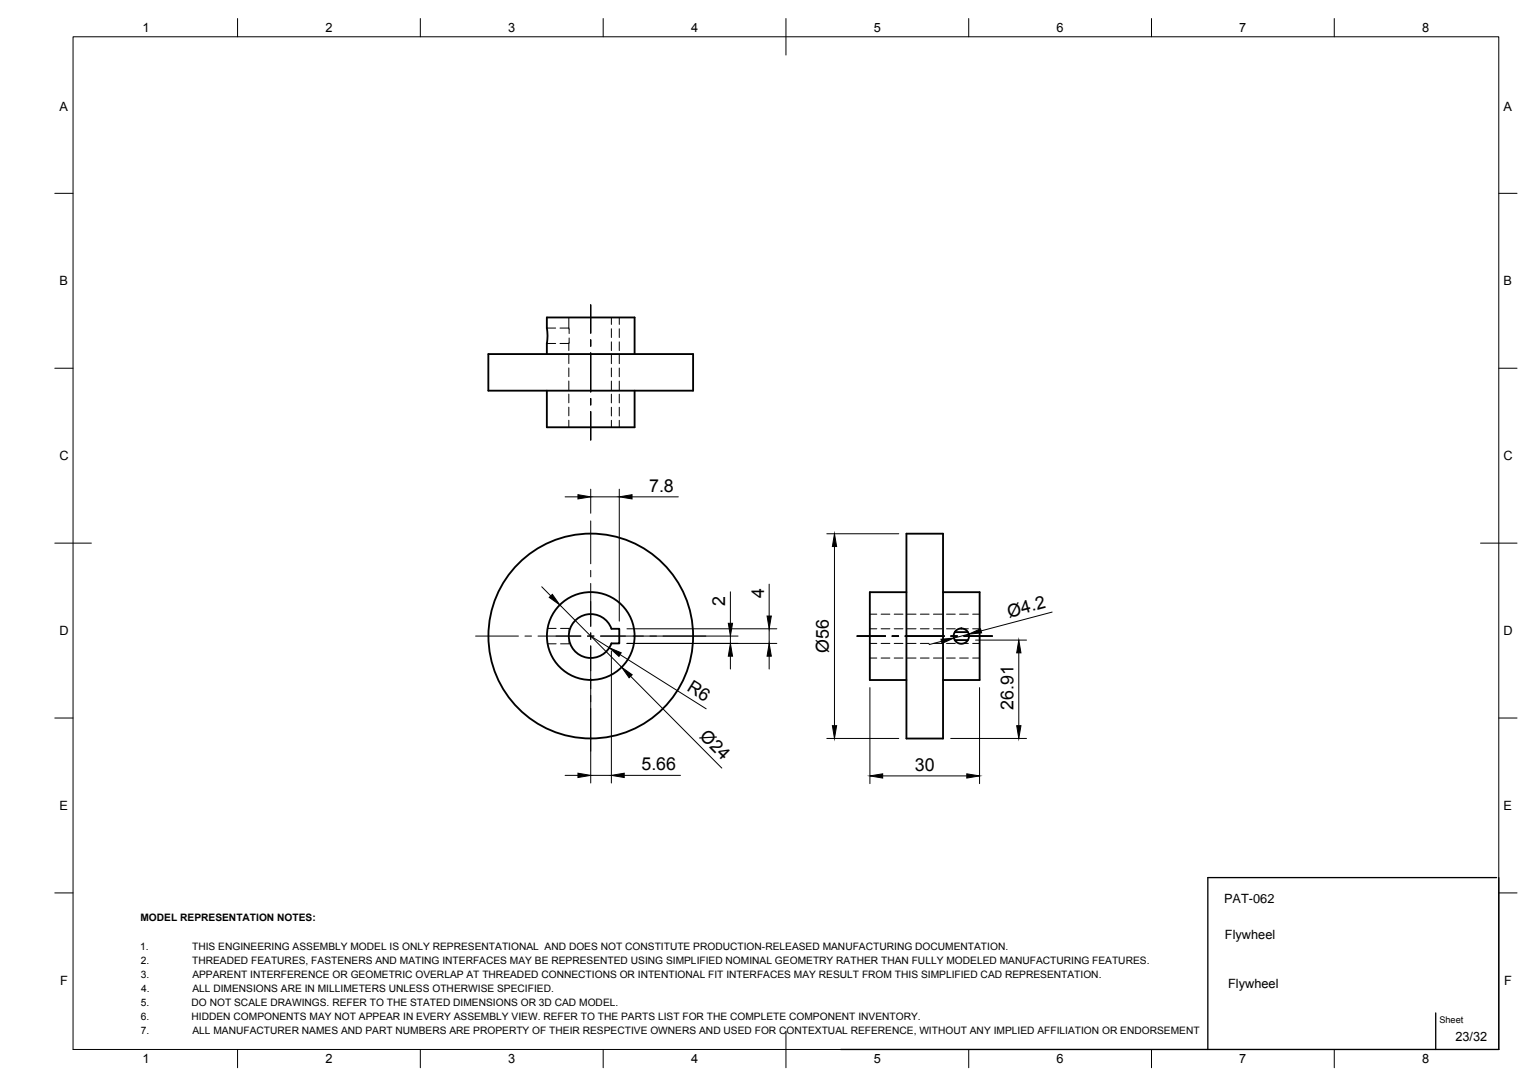
ISO-10303-21;
HEADER;
/* Generated by software containing ST-Developer
 * from STEP Tools, Inc. (www.steptools.com) 
 */

FILE_DESCRIPTION(
/* description */ ('Jaw-coupled motor to shaft test stand'),
/* implementation_level */ '2;1');

FILE_NAME(
/* name */ 'Flywheel.step',
/* time_stamp */ '2026-10-27T10:46:06-07:00',
/* author */ (''),
/* organization */ (''),
/* preprocessor_version */ 'ST-DEVELOPER v20.2',
/* originating_system */ 'Autodesk Translation Framework v15.17.0.0',
/* authorisation */ '');

FILE_SCHEMA (('AUTOMOTIVE_DESIGN { 1 0 10303 214 3 1 1 }'));
ENDSEC;

DATA;
#10=MECHANICAL_DESIGN_GEOMETRIC_PRESENTATION_REPRESENTATION('',(#362),#19361);
#255=B_SPLINE_CURVE_WITH_KNOTS('',3,(#16957,#16958,#16959,#16960,#16961,
#16962,#16963,#16964,#16965,#16966),.UNSPECIFIED.,.F.,.F.,(4,2,2,2,4),(0.847831445683403,
0.87827457693095,0.958092875386316,1.03791117384168,1.06835430508923),
 .UNSPECIFIED.);
#256=B_SPLINE_CURVE_WITH_KNOTS('',3,(#16972,#16973,#16974,#16975,#16976,
#16977,#16978,#16979,#16980,#16981,#16982,#16983,#16984,#16985,#16986,#16987,
#16988,#16989),.UNSPECIFIED.,.F.,.F.,(4,2,2,2,2,2,2,2,4),(0.,0.0792812130427884,
0.158562426085577,0.237841058284634,0.317119690483692,0.396398322682749,
0.475676954881807,0.554958167924595,0.634239380967384),.UNSPECIFIED.);
#257=B_SPLINE_CURVE_WITH_KNOTS('',3,(#16990,#16991,#16992,#16993,#16994,
#16995,#16996,#16997,#16998,#16999,#17000,#17001,#17002,#17003,#17004,#17005,
#17006,#17007),.UNSPECIFIED.,.F.,.F.,(4,2,2,2,2,2,2,2,4),(0.634239380967384,
0.713520594010172,0.792801807052961,0.872080439252018,0.951359071451076,
1.03063770365013,1.10991633584919,1.18919754889198,1.26847876193477),
 .UNSPECIFIED.);
#258=B_SPLINE_CURVE_WITH_KNOTS('',3,(#17010,#17011,#17012,#17013,#17014,
#17015,#17016,#17017,#17018,#17019),.UNSPECIFIED.,.F.,.F.,(4,2,2,2,4),(0.209102862092526,
0.239545993340073,0.319364291795439,0.399182590250804,0.429625721498351),
 .UNSPECIFIED.);
#297=SHAPE_REPRESENTATION_RELATIONSHIP('SRR','None',#19513,#329);
#329=ADVANCED_BREP_SHAPE_REPRESENTATION('',(#393),#19349);
#362=STYLED_ITEM('',(#19760),#393);
#393=MANIFOLD_SOLID_BREP('Body1',#11008);
#489=FACE_BOUND('',#1956,.T.);
#490=FACE_BOUND('',#1958,.T.);
#491=FACE_BOUND('',#1960,.T.);
#492=FACE_BOUND('',#1962,.T.);
#493=FACE_BOUND('',#1965,.T.);
#494=FACE_BOUND('',#1968,.T.);
#666=PLANE('',#11782);
#667=PLANE('',#11787);
#668=PLANE('',#11788);
#669=PLANE('',#11789);
#670=PLANE('',#11790);
#671=PLANE('',#11791);
#672=PLANE('',#11796);
#673=PLANE('',#11799);
#674=PLANE('',#11806);
#1243=FACE_OUTER_BOUND('',#1949,.T.);
#1244=FACE_OUTER_BOUND('',#1950,.T.);
#1245=FACE_OUTER_BOUND('',#1951,.T.);
#1246=FACE_OUTER_BOUND('',#1952,.T.);
#1247=FACE_OUTER_BOUND('',#1953,.T.);
#1248=FACE_OUTER_BOUND('',#1954,.T.);
#1249=FACE_OUTER_BOUND('',#1955,.T.);
#1250=FACE_OUTER_BOUND('',#1957,.T.);
#1251=FACE_OUTER_BOUND('',#1959,.T.);
#1252=FACE_OUTER_BOUND('',#1961,.T.);
#1253=FACE_OUTER_BOUND('',#1963,.T.);
#1254=FACE_OUTER_BOUND('',#1964,.T.);
#1255=FACE_OUTER_BOUND('',#1966,.T.);
#1256=FACE_OUTER_BOUND('',#1967,.T.);
#1949=EDGE_LOOP('',(#8286,#8287));
#1950=EDGE_LOOP('',(#8288,#8289,#8290,#8291,#8292,#8293,#8294,#8295,#8296));
#1951=EDGE_LOOP('',(#8297,#8298,#8299));
#1952=EDGE_LOOP('',(#8300,#8301,#8302,#8303));
#1953=EDGE_LOOP('',(#8304,#8305,#8306,#8307));
#1954=EDGE_LOOP('',(#8308,#8309,#8310,#8311));
#1955=EDGE_LOOP('',(#8312));
#1956=EDGE_LOOP('',(#8313,#8314,#8315,#8316));
#1957=EDGE_LOOP('',(#8317,#8318,#8319,#8320));
#1958=EDGE_LOOP('',(#8321,#8322,#8323,#8324));
#1959=EDGE_LOOP('',(#8325));
#1960=EDGE_LOOP('',(#8326));
#1961=EDGE_LOOP('',(#8327));
#1962=EDGE_LOOP('',(#8328));
#1963=EDGE_LOOP('',(#8329,#8330,#8331,#8332));
#1964=EDGE_LOOP('',(#8333,#8334,#8335,#8336));
#1965=EDGE_LOOP('',(#8337,#8338));
#1966=EDGE_LOOP('',(#8339,#8340,#8341,#8342));
#1967=EDGE_LOOP('',(#8343));
#1968=EDGE_LOOP('',(#8344,#8345,#8346,#8347));
#2682=LINE('',#16953,#3835);
#2683=LINE('',#16970,#3836);
#2684=LINE('',#17021,#3837);
#2685=LINE('',#17025,#3838);
#2686=LINE('',#17027,#3839);
#2687=LINE('',#17029,#3840);
#2688=LINE('',#17030,#3841);
#2689=LINE('',#17033,#3842);
#2690=LINE('',#17035,#3843);
#2691=LINE('',#17036,#3844);
#2692=LINE('',#17039,#3845);
#2693=LINE('',#17041,#3846);
#2694=LINE('',#17042,#3847);
#2695=LINE('',#17060,#3848);
#2696=LINE('',#17063,#3849);
#2697=LINE('',#17066,#3850);
#3835=VECTOR('',#13467,1.);
#3836=VECTOR('',#13474,0.21);
#3837=VECTOR('',#13479,1.);
#3838=VECTOR('',#13482,1.);
#3839=VECTOR('',#13483,1.);
#3840=VECTOR('',#13484,1.);
#3841=VECTOR('',#13485,1.);
#3842=VECTOR('',#13488,1.);
#3843=VECTOR('',#13489,1.);
#3844=VECTOR('',#13490,1.);
#3845=VECTOR('',#13493,1.);
#3846=VECTOR('',#13494,1.);
#3847=VECTOR('',#13495,1.);
#3848=VECTOR('',#13520,2.8);
#3849=VECTOR('',#13523,1.2);
#3850=VECTOR('',#13528,1.2);
#4816=CIRCLE('',#11783,0.21);
#4817=CIRCLE('',#11785,0.21);
#4818=CIRCLE('',#11786,0.21);
#4819=CIRCLE('',#11792,1.2);
#4820=CIRCLE('',#11793,0.6);
#4821=CIRCLE('',#11795,0.6);
#4822=CIRCLE('',#11797,2.8);
#4823=CIRCLE('',#11798,1.2);
#4824=CIRCLE('',#11800,2.8);
#4825=CIRCLE('',#11801,1.2);
#4826=CIRCLE('',#11804,1.2);
#5262=VERTEX_POINT('',#16951);
#5263=VERTEX_POINT('',#16952);
#5264=VERTEX_POINT('',#16956);
#5265=VERTEX_POINT('',#16967);
#5266=VERTEX_POINT('',#16969);
#5267=VERTEX_POINT('',#16971);
#5268=VERTEX_POINT('',#17008);
#5269=VERTEX_POINT('',#17023);
#5270=VERTEX_POINT('',#17024);
#5271=VERTEX_POINT('',#17026);
#5272=VERTEX_POINT('',#17028);
#5273=VERTEX_POINT('',#17032);
#5274=VERTEX_POINT('',#17034);
#5275=VERTEX_POINT('',#17038);
#5276=VERTEX_POINT('',#17040);
#5277=VERTEX_POINT('',#17044);
#5278=VERTEX_POINT('',#17050);
#5279=VERTEX_POINT('',#17052);
#5280=VERTEX_POINT('',#17055);
#5281=VERTEX_POINT('',#17057);
#5282=VERTEX_POINT('',#17062);
#6354=EDGE_CURVE('',#5262,#5263,#2682,.T.);
#6355=EDGE_CURVE('',#5262,#5263,#4816,.T.);
#6356=EDGE_CURVE('',#5264,#5262,#255,.T.);
#6357=EDGE_CURVE('',#5265,#5264,#4817,.T.);
#6358=EDGE_CURVE('',#5265,#5266,#2683,.T.);
#6359=EDGE_CURVE('',#5267,#5266,#256,.T.);
#6360=EDGE_CURVE('',#5266,#5267,#257,.T.);
#6361=EDGE_CURVE('',#5268,#5265,#4818,.T.);
#6362=EDGE_CURVE('',#5263,#5268,#258,.T.);
#6363=EDGE_CURVE('',#5268,#5264,#2684,.T.);
#6364=EDGE_CURVE('',#5269,#5270,#2685,.T.);
#6365=EDGE_CURVE('',#5269,#5271,#2686,.T.);
#6366=EDGE_CURVE('',#5272,#5271,#2687,.T.);
#6367=EDGE_CURVE('',#5270,#5272,#2688,.T.);
#6368=EDGE_CURVE('',#5273,#5269,#2689,.T.);
#6369=EDGE_CURVE('',#5273,#5274,#2690,.T.);
#6370=EDGE_CURVE('',#5271,#5274,#2691,.T.);
#6371=EDGE_CURVE('',#5275,#5273,#2692,.T.);
#6372=EDGE_CURVE('',#5276,#5275,#2693,.T.);
#6373=EDGE_CURVE('',#5274,#5276,#2694,.T.);
#6374=EDGE_CURVE('',#5277,#5277,#4819,.T.);
#6375=EDGE_CURVE('',#5276,#5272,#4820,.T.);
#6376=EDGE_CURVE('',#5275,#5270,#4821,.T.);
#6377=EDGE_CURVE('',#5278,#5278,#4822,.T.);
#6378=EDGE_CURVE('',#5279,#5279,#4823,.T.);
#6379=EDGE_CURVE('',#5280,#5280,#4824,.T.);
#6380=EDGE_CURVE('',#5281,#5281,#4825,.T.);
#6381=EDGE_CURVE('',#5278,#5280,#2695,.T.);
#6382=EDGE_CURVE('',#5281,#5282,#2696,.T.);
#6383=EDGE_CURVE('',#5282,#5282,#4826,.T.);
#6384=EDGE_CURVE('',#5277,#5279,#2697,.T.);
#8286=ORIENTED_EDGE('',*,*,#6354,.F.);
#8287=ORIENTED_EDGE('',*,*,#6355,.T.);
#8288=ORIENTED_EDGE('',*,*,#6356,.F.);
#8289=ORIENTED_EDGE('',*,*,#6357,.F.);
#8290=ORIENTED_EDGE('',*,*,#6358,.T.);
#8291=ORIENTED_EDGE('',*,*,#6359,.F.);
#8292=ORIENTED_EDGE('',*,*,#6360,.F.);
#8293=ORIENTED_EDGE('',*,*,#6358,.F.);
#8294=ORIENTED_EDGE('',*,*,#6361,.F.);
#8295=ORIENTED_EDGE('',*,*,#6362,.F.);
#8296=ORIENTED_EDGE('',*,*,#6355,.F.);
#8297=ORIENTED_EDGE('',*,*,#6363,.F.);
#8298=ORIENTED_EDGE('',*,*,#6361,.T.);
#8299=ORIENTED_EDGE('',*,*,#6357,.T.);
#8300=ORIENTED_EDGE('',*,*,#6364,.F.);
#8301=ORIENTED_EDGE('',*,*,#6365,.T.);
#8302=ORIENTED_EDGE('',*,*,#6366,.F.);
#8303=ORIENTED_EDGE('',*,*,#6367,.F.);
#8304=ORIENTED_EDGE('',*,*,#6368,.F.);
#8305=ORIENTED_EDGE('',*,*,#6369,.T.);
#8306=ORIENTED_EDGE('',*,*,#6370,.F.);
#8307=ORIENTED_EDGE('',*,*,#6365,.F.);
#8308=ORIENTED_EDGE('',*,*,#6371,.F.);
#8309=ORIENTED_EDGE('',*,*,#6372,.F.);
#8310=ORIENTED_EDGE('',*,*,#6373,.F.);
#8311=ORIENTED_EDGE('',*,*,#6369,.F.);
#8312=ORIENTED_EDGE('',*,*,#6374,.T.);
#8313=ORIENTED_EDGE('',*,*,#6366,.T.);
#8314=ORIENTED_EDGE('',*,*,#6370,.T.);
#8315=ORIENTED_EDGE('',*,*,#6373,.T.);
#8316=ORIENTED_EDGE('',*,*,#6375,.T.);
#8317=ORIENTED_EDGE('',*,*,#6367,.T.);
#8318=ORIENTED_EDGE('',*,*,#6375,.F.);
#8319=ORIENTED_EDGE('',*,*,#6372,.T.);
#8320=ORIENTED_EDGE('',*,*,#6376,.T.);
#8321=ORIENTED_EDGE('',*,*,#6362,.T.);
#8322=ORIENTED_EDGE('',*,*,#6363,.T.);
#8323=ORIENTED_EDGE('',*,*,#6356,.T.);
#8324=ORIENTED_EDGE('',*,*,#6354,.T.);
#8325=ORIENTED_EDGE('',*,*,#6377,.T.);
#8326=ORIENTED_EDGE('',*,*,#6378,.F.);
#8327=ORIENTED_EDGE('',*,*,#6379,.F.);
#8328=ORIENTED_EDGE('',*,*,#6380,.F.);
#8329=ORIENTED_EDGE('',*,*,#6377,.F.);
#8330=ORIENTED_EDGE('',*,*,#6381,.T.);
#8331=ORIENTED_EDGE('',*,*,#6379,.T.);
#8332=ORIENTED_EDGE('',*,*,#6381,.F.);
#8333=ORIENTED_EDGE('',*,*,#6380,.T.);
#8334=ORIENTED_EDGE('',*,*,#6382,.T.);
#8335=ORIENTED_EDGE('',*,*,#6383,.T.);
#8336=ORIENTED_EDGE('',*,*,#6382,.F.);
#8337=ORIENTED_EDGE('',*,*,#6359,.T.);
#8338=ORIENTED_EDGE('',*,*,#6360,.T.);
#8339=ORIENTED_EDGE('',*,*,#6374,.F.);
#8340=ORIENTED_EDGE('',*,*,#6384,.T.);
#8341=ORIENTED_EDGE('',*,*,#6378,.T.);
#8342=ORIENTED_EDGE('',*,*,#6384,.F.);
#8343=ORIENTED_EDGE('',*,*,#6383,.F.);
#8344=ORIENTED_EDGE('',*,*,#6364,.T.);
#8345=ORIENTED_EDGE('',*,*,#6376,.F.);
#8346=ORIENTED_EDGE('',*,*,#6371,.T.);
#8347=ORIENTED_EDGE('',*,*,#6368,.T.);
#10333=CYLINDRICAL_SURFACE('',#11784,0.21);
#10334=CYLINDRICAL_SURFACE('',#11794,0.6);
#10335=CYLINDRICAL_SURFACE('',#11802,2.8);
#10336=CYLINDRICAL_SURFACE('',#11803,1.2);
#10337=CYLINDRICAL_SURFACE('',#11805,1.2);
#10585=ADVANCED_FACE('',(#1243),#666,.T.);
#10586=ADVANCED_FACE('',(#1244),#10333,.F.);
#10587=ADVANCED_FACE('',(#1245),#667,.T.);
#10588=ADVANCED_FACE('',(#1246),#668,.F.);
#10589=ADVANCED_FACE('',(#1247),#669,.F.);
#10590=ADVANCED_FACE('',(#1248),#670,.F.);
#10591=ADVANCED_FACE('',(#1249,#489),#671,.T.);
#10592=ADVANCED_FACE('',(#1250,#490),#10334,.F.);
#10593=ADVANCED_FACE('',(#1251,#491),#672,.T.);
#10594=ADVANCED_FACE('',(#1252,#492),#673,.F.);
#10595=ADVANCED_FACE('',(#1253),#10335,.T.);
#10596=ADVANCED_FACE('',(#1254,#493),#10336,.T.);
#10597=ADVANCED_FACE('',(#1255),#10337,.T.);
#10598=ADVANCED_FACE('',(#1256,#494),#674,.F.);
#11008=CLOSED_SHELL('',(#10585,#10586,#10587,#10588,#10589,#10590,#10591,
#10592,#10593,#10594,#10595,#10596,#10597,#10598));
#11781=AXIS2_PLACEMENT_3D('',#16949,#13463,#13464);
#11782=AXIS2_PLACEMENT_3D('',#16950,#13465,#13466);
#11783=AXIS2_PLACEMENT_3D('',#16954,#13468,#13469);
#11784=AXIS2_PLACEMENT_3D('',#16955,#13470,#13471);
#11785=AXIS2_PLACEMENT_3D('',#16968,#13472,#13473);
#11786=AXIS2_PLACEMENT_3D('',#17009,#13475,#13476);
#11787=AXIS2_PLACEMENT_3D('',#17020,#13477,#13478);
#11788=AXIS2_PLACEMENT_3D('',#17022,#13480,#13481);
#11789=AXIS2_PLACEMENT_3D('',#17031,#13486,#13487);
#11790=AXIS2_PLACEMENT_3D('',#17037,#13491,#13492);
#11791=AXIS2_PLACEMENT_3D('',#17043,#13496,#13497);
#11792=AXIS2_PLACEMENT_3D('',#17045,#13498,#13499);
#11793=AXIS2_PLACEMENT_3D('',#17046,#13500,#13501);
#11794=AXIS2_PLACEMENT_3D('',#17047,#13502,#13503);
#11795=AXIS2_PLACEMENT_3D('',#17048,#13504,#13505);
#11796=AXIS2_PLACEMENT_3D('',#17049,#13506,#13507);
#11797=AXIS2_PLACEMENT_3D('',#17051,#13508,#13509);
#11798=AXIS2_PLACEMENT_3D('',#17053,#13510,#13511);
#11799=AXIS2_PLACEMENT_3D('',#17054,#13512,#13513);
#11800=AXIS2_PLACEMENT_3D('',#17056,#13514,#13515);
#11801=AXIS2_PLACEMENT_3D('',#17058,#13516,#13517);
#11802=AXIS2_PLACEMENT_3D('',#17059,#13518,#13519);
#11803=AXIS2_PLACEMENT_3D('',#17061,#13521,#13522);
#11804=AXIS2_PLACEMENT_3D('',#17064,#13524,#13525);
#11805=AXIS2_PLACEMENT_3D('',#17065,#13526,#13527);
#11806=AXIS2_PLACEMENT_3D('',#17067,#13529,#13530);
#13463=DIRECTION('axis',(0.,0.,1.));
#13464=DIRECTION('refdir',(1.,0.,0.));
#13465=DIRECTION('center_axis',(0.,0.,1.));
#13466=DIRECTION('ref_axis',(1.,0.,0.));
#13467=DIRECTION('',(0.,1.,0.));
#13468=DIRECTION('center_axis',(0.,0.,1.));
#13469=DIRECTION('ref_axis',(1.,0.,0.));
#13470=DIRECTION('center_axis',(0.,0.,1.));
#13471=DIRECTION('ref_axis',(1.,0.,0.));
#13472=DIRECTION('center_axis',(0.,0.,1.));
#13473=DIRECTION('ref_axis',(1.,0.,0.));
#13474=DIRECTION('',(0.,0.,1.));
#13475=DIRECTION('center_axis',(0.,0.,1.));
#13476=DIRECTION('ref_axis',(1.,0.,0.));
#13477=DIRECTION('center_axis',(0.,0.,1.));
#13478=DIRECTION('ref_axis',(1.,0.,0.));
#13479=DIRECTION('',(0.,-1.,0.));
#13480=DIRECTION('center_axis',(-1.,0.,0.));
#13481=DIRECTION('ref_axis',(0.,0.,1.));
#13482=DIRECTION('',(0.,0.,1.));
#13483=DIRECTION('',(0.,1.,0.));
#13484=DIRECTION('',(0.,0.,-1.));
#13485=DIRECTION('',(0.,1.,0.));
#13486=DIRECTION('center_axis',(0.,0.,-1.));
#13487=DIRECTION('ref_axis',(-1.,0.,0.));
#13488=DIRECTION('',(-1.,0.,0.));
#13489=DIRECTION('',(0.,1.,0.));
#13490=DIRECTION('',(1.,0.,0.));
#13491=DIRECTION('center_axis',(1.,0.,0.));
#13492=DIRECTION('ref_axis',(0.,0.,-1.));
#13493=DIRECTION('',(0.,0.,-1.));
#13494=DIRECTION('',(0.,-1.,0.));
#13495=DIRECTION('',(0.,0.,1.));
#13496=DIRECTION('center_axis',(0.,1.,0.));
#13497=DIRECTION('ref_axis',(1.,0.,0.));
#13498=DIRECTION('center_axis',(0.,1.,0.));
#13499=DIRECTION('ref_axis',(1.,0.,0.));
#13500=DIRECTION('center_axis',(0.,-1.,0.));
#13501=DIRECTION('ref_axis',(1.,0.,0.));
#13502=DIRECTION('center_axis',(0.,1.,0.));
#13503=DIRECTION('ref_axis',(-1.83697019872103E-16,0.,1.));
#13504=DIRECTION('center_axis',(0.,-1.,0.));
#13505=DIRECTION('ref_axis',(1.,0.,0.));
#13506=DIRECTION('center_axis',(0.,1.,0.));
#13507=DIRECTION('ref_axis',(1.,0.,0.));
#13508=DIRECTION('center_axis',(0.,1.,0.));
#13509=DIRECTION('ref_axis',(1.,0.,0.));
#13510=DIRECTION('center_axis',(0.,1.,0.));
#13511=DIRECTION('ref_axis',(1.,0.,0.));
#13512=DIRECTION('center_axis',(0.,1.,0.));
#13513=DIRECTION('ref_axis',(1.,0.,0.));
#13514=DIRECTION('center_axis',(0.,1.,0.));
#13515=DIRECTION('ref_axis',(1.,0.,0.));
#13516=DIRECTION('center_axis',(0.,-1.,0.));
#13517=DIRECTION('ref_axis',(1.,0.,0.));
#13518=DIRECTION('center_axis',(0.,1.,0.));
#13519=DIRECTION('ref_axis',(1.,0.,0.));
#13520=DIRECTION('',(0.,-1.,0.));
#13521=DIRECTION('center_axis',(0.,1.,0.));
#13522=DIRECTION('ref_axis',(1.,0.,0.));
#13523=DIRECTION('',(0.,-1.,0.));
#13524=DIRECTION('center_axis',(0.,1.,0.));
#13525=DIRECTION('ref_axis',(1.,0.,0.));
#13526=DIRECTION('center_axis',(0.,1.,0.));
#13527=DIRECTION('ref_axis',(1.,0.,0.));
#13528=DIRECTION('',(0.,-1.,0.));
#13529=DIRECTION('center_axis',(0.,1.,0.));
#13530=DIRECTION('ref_axis',(1.,0.,0.));
#16949=CARTESIAN_POINT('',(0.,0.,0.));
#16950=CARTESIAN_POINT('Origin',(0.,9.5,4.81));
#16951=CARTESIAN_POINT('',(0.109087121146358,9.32055641555074,4.81));
#16952=CARTESIAN_POINT('',(0.109087121146358,9.67944358444926,4.81));
#16953=CARTESIAN_POINT('',(0.109087121146358,9.,4.81));
#16954=CARTESIAN_POINT('Origin',(0.,9.5,4.81));
#16955=CARTESIAN_POINT('Origin',(0.,9.5,4.81));
#16956=CARTESIAN_POINT('',(-0.109087121146358,9.32055641555074,4.81));
#16957=CARTESIAN_POINT('Ctrl Pts',(-0.109087121146358,9.32055641555074,
4.81));
#16958=CARTESIAN_POINT('Ctrl Pts',(-0.100058962329436,9.31506802844783,
4.81166924721117));
#16959=CARTESIAN_POINT('Ctrl Pts',(-0.0905297208284663,9.31021510111871,
4.81321436338553));
#16960=CARTESIAN_POINT('Ctrl Pts',(-0.0548356965671429,9.29536302924048,
4.818057680137));
#16961=CARTESIAN_POINT('Ctrl Pts',(-0.026606099485122,9.29,4.82));
#16962=CARTESIAN_POINT('Ctrl Pts',(0.0266060994851219,9.29,4.82));
#16963=CARTESIAN_POINT('Ctrl Pts',(0.0548356965671429,9.29536302924048,
4.818057680137));
#16964=CARTESIAN_POINT('Ctrl Pts',(0.0905297208284663,9.31021510111871,
4.81321436338553));
#16965=CARTESIAN_POINT('Ctrl Pts',(0.100058962329435,9.31506802844783,4.81166924721117));
#16966=CARTESIAN_POINT('Ctrl Pts',(0.109087121146358,9.32055641555074,4.81));
#16967=CARTESIAN_POINT('',(-0.21,9.5,4.81));
#16968=CARTESIAN_POINT('Origin',(0.,9.5,4.81));
#16969=CARTESIAN_POINT('',(-0.21,9.5,5.40148212005091));
#16970=CARTESIAN_POINT('',(-0.21,9.5,4.81));
#16971=CARTESIAN_POINT('',(0.21,9.5,5.40148212005091));
#16972=CARTESIAN_POINT('Ctrl Pts',(0.21,9.5,5.40148212005091));
#16973=CARTESIAN_POINT('Ctrl Pts',(0.21,9.47357292898574,5.40148212005091));
#16974=CARTESIAN_POINT('Ctrl Pts',(0.204707379175837,9.44542244591134,5.40246056146673));
#16975=CARTESIAN_POINT('Ctrl Pts',(0.183259409780015,9.39369943044444,5.40597389417424));
#16976=CARTESIAN_POINT('Ctrl Pts',(0.167106958412512,9.37012211031416,5.40845578531258));
#16977=CARTESIAN_POINT('Ctrl Pts',(0.129878495645339,9.33289364754699,5.4130982535617));
#16978=CARTESIAN_POINT('Ctrl Pts',(0.106300916040875,9.31674072098398,5.41556345497295));
#16979=CARTESIAN_POINT('Ctrl Pts',(0.0545770066794462,9.29529240674315,
5.41903845223025));
#16980=CARTESIAN_POINT('Ctrl Pts',(0.0264262107330192,9.29,5.42));
#16981=CARTESIAN_POINT('Ctrl Pts',(-0.0264262107330192,9.29,5.42));
#16982=CARTESIAN_POINT('Ctrl Pts',(-0.0545770066794462,9.29529240674315,
5.41903845223025));
#16983=CARTESIAN_POINT('Ctrl Pts',(-0.106300916040875,9.31674072098398,
5.41556345497295));
#16984=CARTESIAN_POINT('Ctrl Pts',(-0.129878495645339,9.33289364754699,
5.4130982535617));
#16985=CARTESIAN_POINT('Ctrl Pts',(-0.167106958412512,9.37012211031416,
5.40845578531258));
#16986=CARTESIAN_POINT('Ctrl Pts',(-0.183259409780015,9.39369943044444,
5.40597389417424));
#16987=CARTESIAN_POINT('Ctrl Pts',(-0.204707379175837,9.44542244591134,
5.40246056146673));
#16988=CARTESIAN_POINT('Ctrl Pts',(-0.21,9.47357292898574,5.40148212005091));
#16989=CARTESIAN_POINT('Ctrl Pts',(-0.21,9.5,5.40148212005091));
#16990=CARTESIAN_POINT('Ctrl Pts',(-0.21,9.5,5.40148212005091));
#16991=CARTESIAN_POINT('Ctrl Pts',(-0.21,9.52642707101426,5.40148212005091));
#16992=CARTESIAN_POINT('Ctrl Pts',(-0.204707379175837,9.55457755408866,
5.40246056146673));
#16993=CARTESIAN_POINT('Ctrl Pts',(-0.183259409780015,9.60630056955556,
5.40597389417424));
#16994=CARTESIAN_POINT('Ctrl Pts',(-0.167106958412512,9.62987788968584,
5.40845578531258));
#16995=CARTESIAN_POINT('Ctrl Pts',(-0.129878495645339,9.66710635245301,
5.4130982535617));
#16996=CARTESIAN_POINT('Ctrl Pts',(-0.106300916040875,9.68325927901602,
5.41556345497295));
#16997=CARTESIAN_POINT('Ctrl Pts',(-0.0545770066794462,9.70470759325685,
5.41903845223025));
#16998=CARTESIAN_POINT('Ctrl Pts',(-0.0264262107330192,9.71,5.42));
#16999=CARTESIAN_POINT('Ctrl Pts',(0.0264262107330191,9.71,5.42));
#17000=CARTESIAN_POINT('Ctrl Pts',(0.0545770066794469,9.70470759325685,
5.41903845223025));
#17001=CARTESIAN_POINT('Ctrl Pts',(0.106300916040875,9.68325927901602,5.41556345497295));
#17002=CARTESIAN_POINT('Ctrl Pts',(0.129878495645339,9.66710635245301,5.4130982535617));
#17003=CARTESIAN_POINT('Ctrl Pts',(0.167106958412512,9.62987788968584,5.40845578531258));
#17004=CARTESIAN_POINT('Ctrl Pts',(0.183259409780016,9.60630056955556,5.40597389417424));
#17005=CARTESIAN_POINT('Ctrl Pts',(0.204707379175837,9.55457755408866,5.40246056146672));
#17006=CARTESIAN_POINT('Ctrl Pts',(0.21,9.52642707101426,5.40148212005091));
#17007=CARTESIAN_POINT('Ctrl Pts',(0.21,9.5,5.40148212005091));
#17008=CARTESIAN_POINT('',(-0.109087121146358,9.67944358444926,4.81));
#17009=CARTESIAN_POINT('Origin',(0.,9.5,4.81));
#17010=CARTESIAN_POINT('Ctrl Pts',(0.109087121146358,9.67944358444926,4.81));
#17011=CARTESIAN_POINT('Ctrl Pts',(0.100058962329434,9.68493197155217,4.81166924721117));
#17012=CARTESIAN_POINT('Ctrl Pts',(0.0905297208284663,9.68978489888129,
4.81321436338553));
#17013=CARTESIAN_POINT('Ctrl Pts',(0.054835696567143,9.70463697075952,4.818057680137));
#17014=CARTESIAN_POINT('Ctrl Pts',(0.026606099485122,9.71,4.82));
#17015=CARTESIAN_POINT('Ctrl Pts',(-0.026606099485122,9.71,4.82));
#17016=CARTESIAN_POINT('Ctrl Pts',(-0.0548356965671429,9.70463697075952,
4.818057680137));
#17017=CARTESIAN_POINT('Ctrl Pts',(-0.0905297208284662,9.68978489888129,
4.81321436338553));
#17018=CARTESIAN_POINT('Ctrl Pts',(-0.100058962329435,9.68493197155217,
4.81166924721117));
#17019=CARTESIAN_POINT('Ctrl Pts',(-0.109087121146358,9.67944358444926,
4.81));
#17020=CARTESIAN_POINT('Origin',(0.,9.5,4.81));
#17021=CARTESIAN_POINT('',(-0.109087121146358,9.,4.81));
#17022=CARTESIAN_POINT('Origin',(-0.2,8.9,3.44));
#17023=CARTESIAN_POINT('',(-0.2,9.,3.44));
#17024=CARTESIAN_POINT('',(-0.2,9.,3.65431457505076));
#17025=CARTESIAN_POINT('',(-0.2,9.,3.83));
#17026=CARTESIAN_POINT('',(-0.2,12.,3.44));
#17027=CARTESIAN_POINT('',(-0.2,8.9,3.44));
#17028=CARTESIAN_POINT('',(-0.2,12.,3.65431457505076));
#17029=CARTESIAN_POINT('',(-0.2,12.,3.83));
#17030=CARTESIAN_POINT('',(-0.2,9.,3.65431457505076));
#17031=CARTESIAN_POINT('Origin',(0.2,8.9,3.44));
#17032=CARTESIAN_POINT('',(0.2,9.,3.44));
#17033=CARTESIAN_POINT('',(0.1,9.,3.44));
#17034=CARTESIAN_POINT('',(0.2,12.,3.44));
#17035=CARTESIAN_POINT('',(0.2,8.9,3.44));
#17036=CARTESIAN_POINT('',(0.1,12.,3.44));
#17037=CARTESIAN_POINT('Origin',(0.2,8.9,4.22));
#17038=CARTESIAN_POINT('',(0.2,9.,3.65431457505076));
#17039=CARTESIAN_POINT('',(0.2,9.,4.22));
#17040=CARTESIAN_POINT('',(0.2,12.,3.65431457505076));
#17041=CARTESIAN_POINT('',(0.2,9.,3.65431457505076));
#17042=CARTESIAN_POINT('',(0.2,12.,4.22));
#17043=CARTESIAN_POINT('Origin',(0.,12.,4.22));
#17044=CARTESIAN_POINT('',(-1.2,12.,4.22));
#17045=CARTESIAN_POINT('Origin',(0.,12.,4.22));
#17046=CARTESIAN_POINT('Origin',(0.,12.,4.22));
#17047=CARTESIAN_POINT('Origin',(0.,9.,4.22));
#17048=CARTESIAN_POINT('Origin',(0.,9.,4.22));
#17049=CARTESIAN_POINT('Origin',(0.,11.,4.22));
#17050=CARTESIAN_POINT('',(-2.8,11.,4.22));
#17051=CARTESIAN_POINT('Origin',(0.,11.,4.22));
#17052=CARTESIAN_POINT('',(-1.2,11.,4.22));
#17053=CARTESIAN_POINT('Origin',(0.,11.,4.22));
#17054=CARTESIAN_POINT('Origin',(0.,10.,4.22));
#17055=CARTESIAN_POINT('',(-2.8,10.,4.22));
#17056=CARTESIAN_POINT('Origin',(0.,10.,4.22));
#17057=CARTESIAN_POINT('',(-1.2,10.,4.22));
#17058=CARTESIAN_POINT('Origin',(0.,10.,4.22));
#17059=CARTESIAN_POINT('Origin',(0.,10.,4.22));
#17060=CARTESIAN_POINT('',(-2.8,10.,4.22));
#17061=CARTESIAN_POINT('Origin',(0.,9.,4.22));
#17062=CARTESIAN_POINT('',(-1.2,9.,4.22));
#17063=CARTESIAN_POINT('',(-1.2,9.,4.22));
#17064=CARTESIAN_POINT('Origin',(0.,9.,4.22));
#17065=CARTESIAN_POINT('Origin',(0.,9.,4.22));
#17066=CARTESIAN_POINT('',(-1.2,9.,4.22));
#17067=CARTESIAN_POINT('Origin',(0.,9.,4.22));
#19311=UNCERTAINTY_MEASURE_WITH_UNIT(LENGTH_MEASURE(0.001),#19362,
'DISTANCE_ACCURACY_VALUE',
'Maximum model space distance between geometric entities at asserted c
onnectivities');
#19323=UNCERTAINTY_MEASURE_WITH_UNIT(LENGTH_MEASURE(0.001),#19362,
'DISTANCE_ACCURACY_VALUE',
'Maximum model space distance between geometric entities at asserted c
onnectivities');
#19349=(
GEOMETRIC_REPRESENTATION_CONTEXT(3)
GLOBAL_UNCERTAINTY_ASSIGNED_CONTEXT((#19311))
GLOBAL_UNIT_ASSIGNED_CONTEXT((#19362,#19364,#19365))
REPRESENTATION_CONTEXT('','3D')
);
#19361=(
GEOMETRIC_REPRESENTATION_CONTEXT(3)
GLOBAL_UNCERTAINTY_ASSIGNED_CONTEXT((#19323))
GLOBAL_UNIT_ASSIGNED_CONTEXT((#19362,#19364,#19365))
REPRESENTATION_CONTEXT('','3D')
);
#19362=(
LENGTH_UNIT()
NAMED_UNIT(*)
SI_UNIT(.CENTI.,.METRE.)
);
#19364=(
NAMED_UNIT(*)
PLANE_ANGLE_UNIT()
SI_UNIT($,.RADIAN.)
);
#19365=(
NAMED_UNIT(*)
SI_UNIT($,.STERADIAN.)
SOLID_ANGLE_UNIT()
);
#19391=SHAPE_DEFINITION_REPRESENTATION(#19455,#19513);
#19455=PRODUCT_DEFINITION_SHAPE('',$,#19551);
#19513=SHAPE_REPRESENTATION('',(#11781),#19349);
#19525=PRODUCT_DEFINITION_CONTEXT('part definition',#19638,'design');
#19551=PRODUCT_DEFINITION('Flywheel','Flywheel',#19588,#19525);
#19588=PRODUCT_DEFINITION_FORMATION('',$,#19665);
#19638=APPLICATION_CONTEXT(
'Core Data for Automotive Mechanical Design Process');
#19639=PRODUCT_CONTEXT('part definition',#19638,'mechanical');
#19665=PRODUCT('Flywheel','Flywheel','Flywheel',(#19639));
#19754=COLOUR_RGB('Off White',0.89,0.88,0.83);
#19755=FILL_AREA_STYLE_COLOUR('',#19754);
#19756=FILL_AREA_STYLE('',(#19755));
#19757=SURFACE_STYLE_FILL_AREA(#19756);
#19758=SURFACE_SIDE_STYLE('',(#19757));
#19759=SURFACE_STYLE_USAGE(.BOTH.,#19758);
#19760=PRESENTATION_STYLE_ASSIGNMENT((#19759));
ENDSEC;
END-ISO-10303-21;
